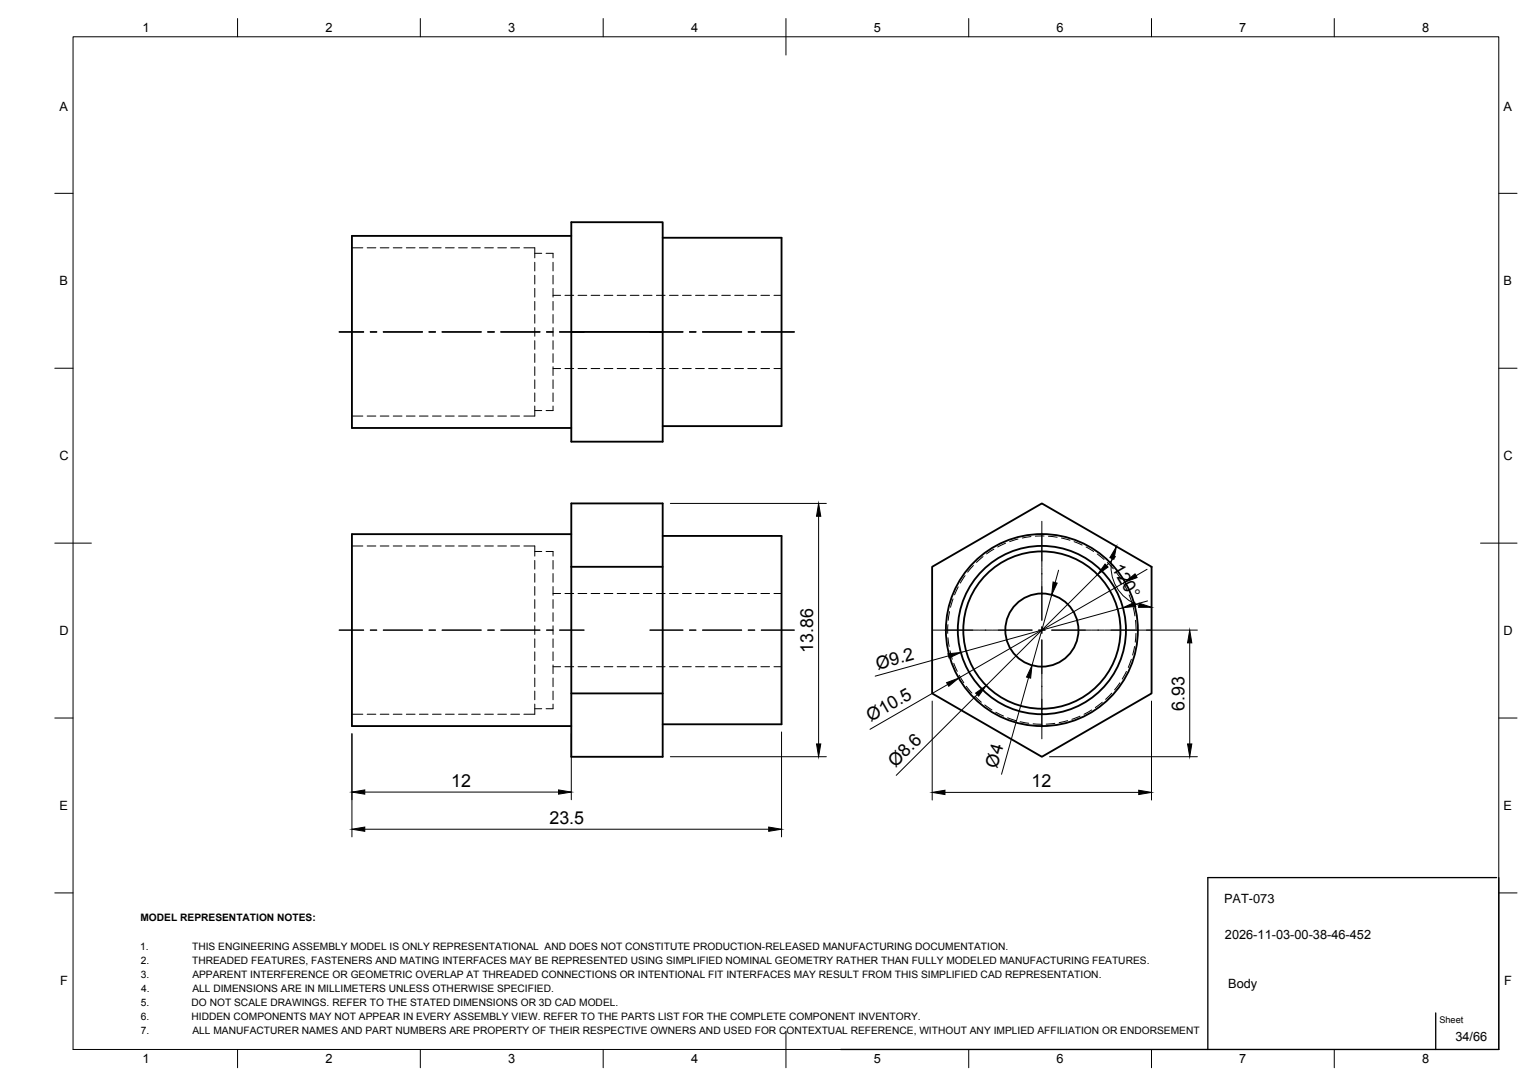
ISO-10303-21;
HEADER;
/* Generated by software containing ST-Developer
 * from STEP Tools, Inc. (www.steptools.com) 
 */

FILE_DESCRIPTION(
/* description */ ('Manual piston pump'),
/* implementation_level */ '2;1');

FILE_NAME(
/* name */ 'Body.step',
/* time_stamp */ '2026-11-02T16:54:23-08:00',
/* author */ (''),
/* organization */ (''),
/* preprocessor_version */ 'ST-DEVELOPER v20.2',
/* originating_system */ 'Autodesk Translation Framework v15.17.0.0',
/* authorisation */ '');

FILE_SCHEMA (('AUTOMOTIVE_DESIGN { 1 0 10303 214 3 1 1 }'));
ENDSEC;

DATA;
#10=MECHANICAL_DESIGN_GEOMETRIC_PRESENTATION_REPRESENTATION('',(#728),#19043);
#594=SHAPE_REPRESENTATION_RELATIONSHIP('SRR','None',#19342,#657);
#657=ADVANCED_BREP_SHAPE_REPRESENTATION('',(#798),#19009);
#728=STYLED_ITEM('',(#19661),#798);
#798=MANIFOLD_SOLID_BREP('Body1',#9514);
#984=FACE_BOUND('',#2371,.T.);
#985=FACE_BOUND('',#2373,.T.);
#986=FACE_BOUND('',#2375,.T.);
#987=FACE_BOUND('',#2383,.T.);
#988=FACE_BOUND('',#2386,.T.);
#989=FACE_BOUND('',#2390,.T.);
#1222=CYLINDRICAL_SURFACE('',#10961,0.43);
#1223=CYLINDRICAL_SURFACE('',#10978,0.46);
#1224=CYLINDRICAL_SURFACE('',#10982,0.525);
#1225=CYLINDRICAL_SURFACE('',#10983,0.515);
#1226=CYLINDRICAL_SURFACE('',#10987,0.2);
#1637=FACE_OUTER_BOUND('',#2369,.T.);
#1638=FACE_OUTER_BOUND('',#2370,.T.);
#1639=FACE_OUTER_BOUND('',#2372,.T.);
#1640=FACE_OUTER_BOUND('',#2374,.T.);
#1641=FACE_OUTER_BOUND('',#2376,.T.);
#1642=FACE_OUTER_BOUND('',#2377,.T.);
#1643=FACE_OUTER_BOUND('',#2378,.T.);
#1644=FACE_OUTER_BOUND('',#2379,.T.);
#1645=FACE_OUTER_BOUND('',#2380,.T.);
#1646=FACE_OUTER_BOUND('',#2381,.T.);
#1647=FACE_OUTER_BOUND('',#2382,.T.);
#1648=FACE_OUTER_BOUND('',#2384,.T.);
#1649=FACE_OUTER_BOUND('',#2385,.T.);
#1650=FACE_OUTER_BOUND('',#2387,.T.);
#1651=FACE_OUTER_BOUND('',#2388,.T.);
#1652=FACE_OUTER_BOUND('',#2389,.T.);
#1653=FACE_OUTER_BOUND('',#2391,.T.);
#2369=EDGE_LOOP('',(#7707,#7708,#7709,#7710));
#2370=EDGE_LOOP('',(#7711));
#2371=EDGE_LOOP('',(#7712));
#2372=EDGE_LOOP('',(#7713,#7714,#7715,#7716,#7717,#7718));
#2373=EDGE_LOOP('',(#7719));
#2374=EDGE_LOOP('',(#7720,#7721,#7722,#7723,#7724,#7725));
#2375=EDGE_LOOP('',(#7726));
#2376=EDGE_LOOP('',(#7727,#7728,#7729,#7730));
#2377=EDGE_LOOP('',(#7731,#7732,#7733,#7734));
#2378=EDGE_LOOP('',(#7735,#7736,#7737,#7738));
#2379=EDGE_LOOP('',(#7739,#7740,#7741,#7742));
#2380=EDGE_LOOP('',(#7743,#7744,#7745,#7746));
#2381=EDGE_LOOP('',(#7747,#7748,#7749,#7750));
#2382=EDGE_LOOP('',(#7751));
#2383=EDGE_LOOP('',(#7752));
#2384=EDGE_LOOP('',(#7753,#7754,#7755,#7756));
#2385=EDGE_LOOP('',(#7757));
#2386=EDGE_LOOP('',(#7758));
#2387=EDGE_LOOP('',(#7759,#7760,#7761,#7762));
#2388=EDGE_LOOP('',(#7763,#7764,#7765,#7766));
#2389=EDGE_LOOP('',(#7767));
#2390=EDGE_LOOP('',(#7768));
#2391=EDGE_LOOP('',(#7769,#7770,#7771,#7772));
#2988=CIRCLE('',#10962,0.43);
#2989=CIRCLE('',#10963,0.43);
#2990=CIRCLE('',#10965,0.2);
#2991=CIRCLE('',#10967,0.525);
#2992=CIRCLE('',#10969,0.515);
#2993=CIRCLE('',#10977,0.46);
#2994=CIRCLE('',#10979,0.46);
#2995=CIRCLE('',#10981,0.525);
#2996=CIRCLE('',#10984,0.515);
#2997=CIRCLE('',#10986,0.2);
#3494=LINE('',#17179,#4098);
#3495=LINE('',#17187,#4099);
#3496=LINE('',#17189,#4100);
#3497=LINE('',#17191,#4101);
#3498=LINE('',#17193,#4102);
#3499=LINE('',#17195,#4103);
#3500=LINE('',#17196,#4104);
#3501=LINE('',#17202,#4105);
#3502=LINE('',#17204,#4106);
#3503=LINE('',#17206,#4107);
#3504=LINE('',#17208,#4108);
#3505=LINE('',#17210,#4109);
#3506=LINE('',#17211,#4110);
#3507=LINE('',#17215,#4111);
#3508=LINE('',#17216,#4112);
#3509=LINE('',#17218,#4113);
#3510=LINE('',#17220,#4114);
#3511=LINE('',#17222,#4115);
#3512=LINE('',#17224,#4116);
#3513=LINE('',#17231,#4117);
#3514=LINE('',#17237,#4118);
#3515=LINE('',#17241,#4119);
#3516=LINE('',#17246,#4120);
#4098=VECTOR('',#13282,0.43);
#4099=VECTOR('',#13291,1.);
#4100=VECTOR('',#13292,1.);
#4101=VECTOR('',#13293,1.);
#4102=VECTOR('',#13294,1.);
#4103=VECTOR('',#13295,1.);
#4104=VECTOR('',#13296,1.);
#4105=VECTOR('',#13301,1.);
#4106=VECTOR('',#13302,1.);
#4107=VECTOR('',#13303,1.);
#4108=VECTOR('',#13304,1.);
#4109=VECTOR('',#13305,1.);
#4110=VECTOR('',#13306,1.);
#4111=VECTOR('',#13311,1.);
#4112=VECTOR('',#13312,1.);
#4113=VECTOR('',#13315,1.);
#4114=VECTOR('',#13318,1.);
#4115=VECTOR('',#13321,1.);
#4116=VECTOR('',#13324,1.);
#4117=VECTOR('',#13333,0.46);
#4118=VECTOR('',#13342,0.525);
#4119=VECTOR('',#13347,0.515);
#4120=VECTOR('',#13354,0.2);
#4838=VERTEX_POINT('',#17176);
#4839=VERTEX_POINT('',#17178);
#4840=VERTEX_POINT('',#17182);
#4841=VERTEX_POINT('',#17185);
#4842=VERTEX_POINT('',#17186);
#4843=VERTEX_POINT('',#17188);
#4844=VERTEX_POINT('',#17190);
#4845=VERTEX_POINT('',#17192);
#4846=VERTEX_POINT('',#17194);
#4847=VERTEX_POINT('',#17197);
#4848=VERTEX_POINT('',#17200);
#4849=VERTEX_POINT('',#17201);
#4850=VERTEX_POINT('',#17203);
#4851=VERTEX_POINT('',#17205);
#4852=VERTEX_POINT('',#17207);
#4853=VERTEX_POINT('',#17209);
#4854=VERTEX_POINT('',#17212);
#4855=VERTEX_POINT('',#17227);
#4856=VERTEX_POINT('',#17230);
#4857=VERTEX_POINT('',#17234);
#4858=VERTEX_POINT('',#17239);
#4859=VERTEX_POINT('',#17243);
#5840=EDGE_CURVE('',#4838,#4838,#2988,.T.);
#5841=EDGE_CURVE('',#4838,#4839,#3494,.T.);
#5842=EDGE_CURVE('',#4839,#4839,#2989,.T.);
#5843=EDGE_CURVE('',#4840,#4840,#2990,.T.);
#5844=EDGE_CURVE('',#4841,#4842,#3495,.T.);
#5845=EDGE_CURVE('',#4842,#4843,#3496,.T.);
#5846=EDGE_CURVE('',#4843,#4844,#3497,.T.);
#5847=EDGE_CURVE('',#4844,#4845,#3498,.T.);
#5848=EDGE_CURVE('',#4845,#4846,#3499,.T.);
#5849=EDGE_CURVE('',#4846,#4841,#3500,.T.);
#5850=EDGE_CURVE('',#4847,#4847,#2991,.T.);
#5851=EDGE_CURVE('',#4848,#4849,#3501,.T.);
#5852=EDGE_CURVE('',#4850,#4848,#3502,.T.);
#5853=EDGE_CURVE('',#4851,#4850,#3503,.T.);
#5854=EDGE_CURVE('',#4852,#4851,#3504,.T.);
#5855=EDGE_CURVE('',#4853,#4852,#3505,.T.);
#5856=EDGE_CURVE('',#4849,#4853,#3506,.T.);
#5857=EDGE_CURVE('',#4854,#4854,#2992,.T.);
#5858=EDGE_CURVE('',#4848,#4841,#3507,.T.);
#5859=EDGE_CURVE('',#4850,#4846,#3508,.T.);
#5860=EDGE_CURVE('',#4851,#4845,#3509,.T.);
#5861=EDGE_CURVE('',#4852,#4844,#3510,.T.);
#5862=EDGE_CURVE('',#4853,#4843,#3511,.T.);
#5863=EDGE_CURVE('',#4849,#4842,#3512,.T.);
#5864=EDGE_CURVE('',#4855,#4855,#2993,.T.);
#5865=EDGE_CURVE('',#4855,#4856,#3513,.T.);
#5866=EDGE_CURVE('',#4856,#4856,#2994,.T.);
#5867=EDGE_CURVE('',#4857,#4857,#2995,.T.);
#5868=EDGE_CURVE('',#4847,#4857,#3514,.T.);
#5869=EDGE_CURVE('',#4858,#4858,#2996,.T.);
#5870=EDGE_CURVE('',#4858,#4854,#3515,.T.);
#5871=EDGE_CURVE('',#4859,#4859,#2997,.T.);
#5872=EDGE_CURVE('',#4859,#4840,#3516,.T.);
#7707=ORIENTED_EDGE('',*,*,#5840,.F.);
#7708=ORIENTED_EDGE('',*,*,#5841,.T.);
#7709=ORIENTED_EDGE('',*,*,#5842,.F.);
#7710=ORIENTED_EDGE('',*,*,#5841,.F.);
#7711=ORIENTED_EDGE('',*,*,#5840,.T.);
#7712=ORIENTED_EDGE('',*,*,#5843,.F.);
#7713=ORIENTED_EDGE('',*,*,#5844,.T.);
#7714=ORIENTED_EDGE('',*,*,#5845,.T.);
#7715=ORIENTED_EDGE('',*,*,#5846,.T.);
#7716=ORIENTED_EDGE('',*,*,#5847,.T.);
#7717=ORIENTED_EDGE('',*,*,#5848,.T.);
#7718=ORIENTED_EDGE('',*,*,#5849,.T.);
#7719=ORIENTED_EDGE('',*,*,#5850,.T.);
#7720=ORIENTED_EDGE('',*,*,#5851,.F.);
#7721=ORIENTED_EDGE('',*,*,#5852,.F.);
#7722=ORIENTED_EDGE('',*,*,#5853,.F.);
#7723=ORIENTED_EDGE('',*,*,#5854,.F.);
#7724=ORIENTED_EDGE('',*,*,#5855,.F.);
#7725=ORIENTED_EDGE('',*,*,#5856,.F.);
#7726=ORIENTED_EDGE('',*,*,#5857,.F.);
#7727=ORIENTED_EDGE('',*,*,#5852,.T.);
#7728=ORIENTED_EDGE('',*,*,#5858,.T.);
#7729=ORIENTED_EDGE('',*,*,#5849,.F.);
#7730=ORIENTED_EDGE('',*,*,#5859,.F.);
#7731=ORIENTED_EDGE('',*,*,#5853,.T.);
#7732=ORIENTED_EDGE('',*,*,#5859,.T.);
#7733=ORIENTED_EDGE('',*,*,#5848,.F.);
#7734=ORIENTED_EDGE('',*,*,#5860,.F.);
#7735=ORIENTED_EDGE('',*,*,#5854,.T.);
#7736=ORIENTED_EDGE('',*,*,#5860,.T.);
#7737=ORIENTED_EDGE('',*,*,#5847,.F.);
#7738=ORIENTED_EDGE('',*,*,#5861,.F.);
#7739=ORIENTED_EDGE('',*,*,#5855,.T.);
#7740=ORIENTED_EDGE('',*,*,#5861,.T.);
#7741=ORIENTED_EDGE('',*,*,#5846,.F.);
#7742=ORIENTED_EDGE('',*,*,#5862,.F.);
#7743=ORIENTED_EDGE('',*,*,#5856,.T.);
#7744=ORIENTED_EDGE('',*,*,#5862,.T.);
#7745=ORIENTED_EDGE('',*,*,#5845,.F.);
#7746=ORIENTED_EDGE('',*,*,#5863,.F.);
#7747=ORIENTED_EDGE('',*,*,#5851,.T.);
#7748=ORIENTED_EDGE('',*,*,#5863,.T.);
#7749=ORIENTED_EDGE('',*,*,#5844,.F.);
#7750=ORIENTED_EDGE('',*,*,#5858,.F.);
#7751=ORIENTED_EDGE('',*,*,#5864,.F.);
#7752=ORIENTED_EDGE('',*,*,#5842,.T.);
#7753=ORIENTED_EDGE('',*,*,#5864,.T.);
#7754=ORIENTED_EDGE('',*,*,#5865,.T.);
#7755=ORIENTED_EDGE('',*,*,#5866,.F.);
#7756=ORIENTED_EDGE('',*,*,#5865,.F.);
#7757=ORIENTED_EDGE('',*,*,#5867,.F.);
#7758=ORIENTED_EDGE('',*,*,#5866,.T.);
#7759=ORIENTED_EDGE('',*,*,#5850,.F.);
#7760=ORIENTED_EDGE('',*,*,#5868,.T.);
#7761=ORIENTED_EDGE('',*,*,#5867,.T.);
#7762=ORIENTED_EDGE('',*,*,#5868,.F.);
#7763=ORIENTED_EDGE('',*,*,#5869,.F.);
#7764=ORIENTED_EDGE('',*,*,#5870,.T.);
#7765=ORIENTED_EDGE('',*,*,#5857,.T.);
#7766=ORIENTED_EDGE('',*,*,#5870,.F.);
#7767=ORIENTED_EDGE('',*,*,#5869,.T.);
#7768=ORIENTED_EDGE('',*,*,#5871,.F.);
#7769=ORIENTED_EDGE('',*,*,#5871,.T.);
#7770=ORIENTED_EDGE('',*,*,#5872,.T.);
#7771=ORIENTED_EDGE('',*,*,#5843,.T.);
#7772=ORIENTED_EDGE('',*,*,#5872,.F.);
#8752=PLANE('',#10964);
#8753=PLANE('',#10966);
#8754=PLANE('',#10968);
#8755=PLANE('',#10970);
#8756=PLANE('',#10971);
#8757=PLANE('',#10972);
#8758=PLANE('',#10973);
#8759=PLANE('',#10974);
#8760=PLANE('',#10975);
#8761=PLANE('',#10976);
#8762=PLANE('',#10980);
#8763=PLANE('',#10985);
#9242=ADVANCED_FACE('',(#1637),#1222,.F.);
#9243=ADVANCED_FACE('',(#1638,#984),#8752,.T.);
#9244=ADVANCED_FACE('',(#1639,#985),#8753,.T.);
#9245=ADVANCED_FACE('',(#1640,#986),#8754,.F.);
#9246=ADVANCED_FACE('',(#1641),#8755,.T.);
#9247=ADVANCED_FACE('',(#1642),#8756,.T.);
#9248=ADVANCED_FACE('',(#1643),#8757,.T.);
#9249=ADVANCED_FACE('',(#1644),#8758,.T.);
#9250=ADVANCED_FACE('',(#1645),#8759,.T.);
#9251=ADVANCED_FACE('',(#1646),#8760,.T.);
#9252=ADVANCED_FACE('',(#1647,#987),#8761,.T.);
#9253=ADVANCED_FACE('',(#1648),#1223,.F.);
#9254=ADVANCED_FACE('',(#1649,#988),#8762,.T.);
#9255=ADVANCED_FACE('',(#1650),#1224,.T.);
#9256=ADVANCED_FACE('',(#1651),#1225,.T.);
#9257=ADVANCED_FACE('',(#1652,#989),#8763,.T.);
#9258=ADVANCED_FACE('',(#1653),#1226,.F.);
#9514=CLOSED_SHELL('',(#9242,#9243,#9244,#9245,#9246,#9247,#9248,#9249,
#9250,#9251,#9252,#9253,#9254,#9255,#9256,#9257,#9258));
#10960=AXIS2_PLACEMENT_3D('',#17174,#13276,#13277);
#10961=AXIS2_PLACEMENT_3D('',#17175,#13278,#13279);
#10962=AXIS2_PLACEMENT_3D('',#17177,#13280,#13281);
#10963=AXIS2_PLACEMENT_3D('',#17180,#13283,#13284);
#10964=AXIS2_PLACEMENT_3D('',#17181,#13285,#13286);
#10965=AXIS2_PLACEMENT_3D('',#17183,#13287,#13288);
#10966=AXIS2_PLACEMENT_3D('',#17184,#13289,#13290);
#10967=AXIS2_PLACEMENT_3D('',#17198,#13297,#13298);
#10968=AXIS2_PLACEMENT_3D('',#17199,#13299,#13300);
#10969=AXIS2_PLACEMENT_3D('',#17213,#13307,#13308);
#10970=AXIS2_PLACEMENT_3D('',#17214,#13309,#13310);
#10971=AXIS2_PLACEMENT_3D('',#17217,#13313,#13314);
#10972=AXIS2_PLACEMENT_3D('',#17219,#13316,#13317);
#10973=AXIS2_PLACEMENT_3D('',#17221,#13319,#13320);
#10974=AXIS2_PLACEMENT_3D('',#17223,#13322,#13323);
#10975=AXIS2_PLACEMENT_3D('',#17225,#13325,#13326);
#10976=AXIS2_PLACEMENT_3D('',#17226,#13327,#13328);
#10977=AXIS2_PLACEMENT_3D('',#17228,#13329,#13330);
#10978=AXIS2_PLACEMENT_3D('',#17229,#13331,#13332);
#10979=AXIS2_PLACEMENT_3D('',#17232,#13334,#13335);
#10980=AXIS2_PLACEMENT_3D('',#17233,#13336,#13337);
#10981=AXIS2_PLACEMENT_3D('',#17235,#13338,#13339);
#10982=AXIS2_PLACEMENT_3D('',#17236,#13340,#13341);
#10983=AXIS2_PLACEMENT_3D('',#17238,#13343,#13344);
#10984=AXIS2_PLACEMENT_3D('',#17240,#13345,#13346);
#10985=AXIS2_PLACEMENT_3D('',#17242,#13348,#13349);
#10986=AXIS2_PLACEMENT_3D('',#17244,#13350,#13351);
#10987=AXIS2_PLACEMENT_3D('',#17245,#13352,#13353);
#13276=DIRECTION('axis',(0.,0.,1.));
#13277=DIRECTION('refdir',(1.,0.,0.));
#13278=DIRECTION('center_axis',(0.,1.,0.));
#13279=DIRECTION('ref_axis',(1.,0.,0.));
#13280=DIRECTION('center_axis',(0.,1.,0.));
#13281=DIRECTION('ref_axis',(1.,0.,0.));
#13282=DIRECTION('',(0.,1.,0.));
#13283=DIRECTION('center_axis',(0.,-1.,0.));
#13284=DIRECTION('ref_axis',(1.,0.,0.));
#13285=DIRECTION('center_axis',(0.,1.,0.));
#13286=DIRECTION('ref_axis',(1.,0.,0.));
#13287=DIRECTION('center_axis',(0.,1.,0.));
#13288=DIRECTION('ref_axis',(1.,0.,0.));
#13289=DIRECTION('center_axis',(0.,1.,0.));
#13290=DIRECTION('ref_axis',(1.,0.,0.));
#13291=DIRECTION('',(0.5,0.,-0.866025403784439));
#13292=DIRECTION('',(-0.5,0.,-0.866025403784439));
#13293=DIRECTION('',(-1.,0.,-1.60246890531964E-16));
#13294=DIRECTION('',(-0.5,0.,0.866025403784439));
#13295=DIRECTION('',(0.5,0.,0.866025403784439));
#13296=DIRECTION('',(1.,0.,1.60246890531964E-16));
#13297=DIRECTION('center_axis',(0.,-1.,0.));
#13298=DIRECTION('ref_axis',(1.,0.,0.));
#13299=DIRECTION('center_axis',(0.,1.,0.));
#13300=DIRECTION('ref_axis',(1.,0.,0.));
#13301=DIRECTION('',(0.5,0.,-0.866025403784439));
#13302=DIRECTION('',(1.,0.,1.60246890531964E-16));
#13303=DIRECTION('',(0.5,0.,0.866025403784439));
#13304=DIRECTION('',(-0.5,0.,0.866025403784439));
#13305=DIRECTION('',(-1.,0.,-1.60246890531964E-16));
#13306=DIRECTION('',(-0.5,0.,-0.866025403784439));
#13307=DIRECTION('center_axis',(0.,-1.,0.));
#13308=DIRECTION('ref_axis',(1.,0.,0.));
#13309=DIRECTION('center_axis',(-1.60246890531964E-16,0.,1.));
#13310=DIRECTION('ref_axis',(1.,0.,1.60246890531964E-16));
#13311=DIRECTION('',(0.,1.,0.));
#13312=DIRECTION('',(0.,1.,0.));
#13313=DIRECTION('center_axis',(-0.866025403784439,0.,0.5));
#13314=DIRECTION('ref_axis',(0.5,0.,0.866025403784439));
#13315=DIRECTION('',(0.,1.,0.));
#13316=DIRECTION('center_axis',(-0.866025403784439,0.,-0.5));
#13317=DIRECTION('ref_axis',(-0.5,0.,0.866025403784439));
#13318=DIRECTION('',(0.,1.,0.));
#13319=DIRECTION('center_axis',(1.60246890531964E-16,0.,-1.));
#13320=DIRECTION('ref_axis',(-1.,0.,-1.60246890531964E-16));
#13321=DIRECTION('',(0.,1.,0.));
#13322=DIRECTION('center_axis',(0.866025403784439,0.,-0.5));
#13323=DIRECTION('ref_axis',(-0.5,0.,-0.866025403784439));
#13324=DIRECTION('',(0.,1.,0.));
#13325=DIRECTION('center_axis',(0.866025403784439,0.,0.5));
#13326=DIRECTION('ref_axis',(0.5,0.,-0.866025403784439));
#13327=DIRECTION('center_axis',(0.,1.,0.));
#13328=DIRECTION('ref_axis',(0.,0.,1.));
#13329=DIRECTION('center_axis',(0.,-1.,0.));
#13330=DIRECTION('ref_axis',(1.,0.,0.));
#13331=DIRECTION('center_axis',(0.,-1.,0.));
#13332=DIRECTION('ref_axis',(1.,0.,0.));
#13333=DIRECTION('',(0.,1.,0.));
#13334=DIRECTION('center_axis',(0.,-1.,0.));
#13335=DIRECTION('ref_axis',(1.,0.,0.));
#13336=DIRECTION('center_axis',(0.,1.,0.));
#13337=DIRECTION('ref_axis',(0.,0.,1.));
#13338=DIRECTION('center_axis',(0.,-1.,0.));
#13339=DIRECTION('ref_axis',(1.,0.,0.));
#13340=DIRECTION('center_axis',(0.,-1.,0.));
#13341=DIRECTION('ref_axis',(1.,0.,0.));
#13342=DIRECTION('',(0.,1.,0.));
#13343=DIRECTION('center_axis',(0.,-1.,0.));
#13344=DIRECTION('ref_axis',(1.,0.,0.));
#13345=DIRECTION('center_axis',(0.,-1.,0.));
#13346=DIRECTION('ref_axis',(1.,0.,0.));
#13347=DIRECTION('',(0.,1.,0.));
#13348=DIRECTION('center_axis',(0.,-1.,0.));
#13349=DIRECTION('ref_axis',(0.,0.,-1.));
#13350=DIRECTION('center_axis',(0.,-1.,0.));
#13351=DIRECTION('ref_axis',(1.,0.,0.));
#13352=DIRECTION('center_axis',(0.,-1.,0.));
#13353=DIRECTION('ref_axis',(1.,0.,0.));
#13354=DIRECTION('',(0.,1.,0.));
#17174=CARTESIAN_POINT('',(0.,0.,0.));
#17175=CARTESIAN_POINT('Origin',(0.,0.6,0.));
#17176=CARTESIAN_POINT('',(-0.43,0.6,5.26598123633362E-17));
#17177=CARTESIAN_POINT('Origin',(0.,0.6,0.));
#17178=CARTESIAN_POINT('',(-0.43,0.7,-5.26598123633362E-17));
#17179=CARTESIAN_POINT('',(-0.43,0.6,5.26598123633362E-17));
#17180=CARTESIAN_POINT('Origin',(0.,0.7,0.));
#17181=CARTESIAN_POINT('Origin',(0.,0.6,0.));
#17182=CARTESIAN_POINT('',(-0.2,0.6,2.44929359829471E-17));
#17183=CARTESIAN_POINT('Origin',(0.,0.6,0.));
#17184=CARTESIAN_POINT('Origin',(0.,0.5,-1.11022302462516E-16));
#17185=CARTESIAN_POINT('',(0.346410161513776,0.5,0.6));
#17186=CARTESIAN_POINT('',(0.692820323027551,0.5,0.));
#17187=CARTESIAN_POINT('',(0.346410161513776,0.5,0.6));
#17188=CARTESIAN_POINT('',(0.346410161513776,0.5,-0.6));
#17189=CARTESIAN_POINT('',(0.692820323027551,0.5,0.));
#17190=CARTESIAN_POINT('',(-0.346410161513775,0.5,-0.6));
#17191=CARTESIAN_POINT('',(0.346410161513776,0.5,-0.6));
#17192=CARTESIAN_POINT('',(-0.692820323027551,0.5,-8.48460190979926E-17));
#17193=CARTESIAN_POINT('',(-0.346410161513775,0.5,-0.6));
#17194=CARTESIAN_POINT('',(-0.346410161513776,0.5,0.6));
#17195=CARTESIAN_POINT('',(-0.692820323027551,0.5,-8.48460190979926E-17));
#17196=CARTESIAN_POINT('',(-0.346410161513776,0.5,0.6));
#17197=CARTESIAN_POINT('',(-0.525,0.5,-6.4293956955236E-17));
#17198=CARTESIAN_POINT('Origin',(0.,0.5,0.));
#17199=CARTESIAN_POINT('Origin',(0.,0.,-1.11022302462516E-16));
#17200=CARTESIAN_POINT('',(0.346410161513776,0.,0.6));
#17201=CARTESIAN_POINT('',(0.692820323027551,0.,0.));
#17202=CARTESIAN_POINT('',(0.346410161513776,0.,0.6));
#17203=CARTESIAN_POINT('',(-0.346410161513776,0.,0.6));
#17204=CARTESIAN_POINT('',(-0.346410161513776,0.,0.6));
#17205=CARTESIAN_POINT('',(-0.692820323027551,0.,-8.48460190979926E-17));
#17206=CARTESIAN_POINT('',(-0.692820323027551,0.,-8.48460190979926E-17));
#17207=CARTESIAN_POINT('',(-0.346410161513775,0.,-0.6));
#17208=CARTESIAN_POINT('',(-0.346410161513775,0.,-0.6));
#17209=CARTESIAN_POINT('',(0.346410161513776,0.,-0.6));
#17210=CARTESIAN_POINT('',(0.346410161513776,0.,-0.6));
#17211=CARTESIAN_POINT('',(0.692820323027551,0.,0.));
#17212=CARTESIAN_POINT('',(-0.515,0.,-6.30693101560887E-17));
#17213=CARTESIAN_POINT('Origin',(0.,0.,0.));
#17214=CARTESIAN_POINT('Origin',(-0.346410161513776,0.,0.6));
#17215=CARTESIAN_POINT('',(0.346410161513776,0.,0.6));
#17216=CARTESIAN_POINT('',(-0.346410161513776,0.,0.6));
#17217=CARTESIAN_POINT('Origin',(-0.692820323027551,0.,-8.48460190979926E-17));
#17218=CARTESIAN_POINT('',(-0.692820323027551,0.,-8.48460190979926E-17));
#17219=CARTESIAN_POINT('Origin',(-0.346410161513775,0.,-0.6));
#17220=CARTESIAN_POINT('',(-0.346410161513775,0.,-0.6));
#17221=CARTESIAN_POINT('Origin',(0.346410161513776,0.,-0.6));
#17222=CARTESIAN_POINT('',(0.346410161513776,0.,-0.6));
#17223=CARTESIAN_POINT('Origin',(0.692820323027551,0.,0.));
#17224=CARTESIAN_POINT('',(0.692820323027551,0.,0.));
#17225=CARTESIAN_POINT('Origin',(0.346410161513776,0.,0.6));
#17226=CARTESIAN_POINT('Origin',(0.46,0.7,0.));
#17227=CARTESIAN_POINT('',(-0.46,0.7,-5.63337527607782E-17));
#17228=CARTESIAN_POINT('Origin',(0.,0.7,0.));
#17229=CARTESIAN_POINT('Origin',(0.,1.2,0.));
#17230=CARTESIAN_POINT('',(-0.46,1.7,-5.63337527607782E-17));
#17231=CARTESIAN_POINT('',(-0.46,1.2,-5.63337527607782E-17));
#17232=CARTESIAN_POINT('Origin',(0.,1.7,0.));
#17233=CARTESIAN_POINT('Origin',(0.525,1.7,0.));
#17234=CARTESIAN_POINT('',(-0.525,1.7,-6.4293956955236E-17));
#17235=CARTESIAN_POINT('Origin',(0.,1.7,0.));
#17236=CARTESIAN_POINT('Origin',(0.,1.1,0.));
#17237=CARTESIAN_POINT('',(-0.525,1.1,-6.4293956955236E-17));
#17238=CARTESIAN_POINT('Origin',(0.,-0.325,0.));
#17239=CARTESIAN_POINT('',(-0.515,-0.65,-6.30693101560887E-17));
#17240=CARTESIAN_POINT('Origin',(0.,-0.65,0.));
#17241=CARTESIAN_POINT('',(-0.515,-0.325,-6.30693101560887E-17));
#17242=CARTESIAN_POINT('Origin',(0.2,-0.65,0.));
#17243=CARTESIAN_POINT('',(-0.2,-0.65,-2.44929359829471E-17));
#17244=CARTESIAN_POINT('Origin',(0.,-0.65,0.));
#17245=CARTESIAN_POINT('Origin',(0.,0.0249999999999999,0.));
#17246=CARTESIAN_POINT('',(-0.2,0.0249999999999999,-2.44929359829471E-17));
#18938=UNCERTAINTY_MEASURE_WITH_UNIT(LENGTH_MEASURE(0.001),#19044,
'DISTANCE_ACCURACY_VALUE',
'Maximum model space distance between geometric entities at asserted c
onnectivities');
#18972=UNCERTAINTY_MEASURE_WITH_UNIT(LENGTH_MEASURE(0.001),#19044,
'DISTANCE_ACCURACY_VALUE',
'Maximum model space distance between geometric entities at asserted c
onnectivities');
#19009=(
GEOMETRIC_REPRESENTATION_CONTEXT(3)
GLOBAL_UNCERTAINTY_ASSIGNED_CONTEXT((#18938))
GLOBAL_UNIT_ASSIGNED_CONTEXT((#19044,#19046,#19047))
REPRESENTATION_CONTEXT('','3D')
);
#19043=(
GEOMETRIC_REPRESENTATION_CONTEXT(3)
GLOBAL_UNCERTAINTY_ASSIGNED_CONTEXT((#18972))
GLOBAL_UNIT_ASSIGNED_CONTEXT((#19044,#19046,#19047))
REPRESENTATION_CONTEXT('','3D')
);
#19044=(
LENGTH_UNIT()
NAMED_UNIT(*)
SI_UNIT(.CENTI.,.METRE.)
);
#19046=(
NAMED_UNIT(*)
PLANE_ANGLE_UNIT()
SI_UNIT($,.RADIAN.)
);
#19047=(
NAMED_UNIT(*)
SI_UNIT($,.STERADIAN.)
SOLID_ANGLE_UNIT()
);
#19084=SHAPE_DEFINITION_REPRESENTATION(#19159,#19342);
#19159=PRODUCT_DEFINITION_SHAPE('',$,#19413);
#19342=SHAPE_REPRESENTATION('',(#10960),#19009);
#19376=PRODUCT_DEFINITION_CONTEXT('part definition',#19588,'design');
#19413=PRODUCT_DEFINITION('2026-11-03-00-38-46-452','Body',#19483,#19376);
#19483=PRODUCT_DEFINITION_FORMATION('',$,#19626);
#19588=APPLICATION_CONTEXT(
'Core Data for Automotive Mechanical Design Process');
#19589=PRODUCT_CONTEXT('part definition',#19588,'mechanical');
#19626=PRODUCT('2026-11-03-00-38-46-452','Body','Body',(#19589));
#19661=PRESENTATION_STYLE_ASSIGNMENT((#19667));
#19667=SURFACE_STYLE_USAGE(.BOTH.,#19673);
#19673=SURFACE_SIDE_STYLE('',(#19679));
#19679=SURFACE_STYLE_FILL_AREA(#19685);
#19685=FILL_AREA_STYLE('CAD Library Painted - Engineering blue',(#19691));
#19691=FILL_AREA_STYLE_COLOUR('CAD Library Painted - Engineering blue',
#19697);
#19697=COLOUR_RGB('CAD Library Painted - Engineering blue',0.12156862745098,
0.356862745098039,0.6);
ENDSEC;
END-ISO-10303-21;
